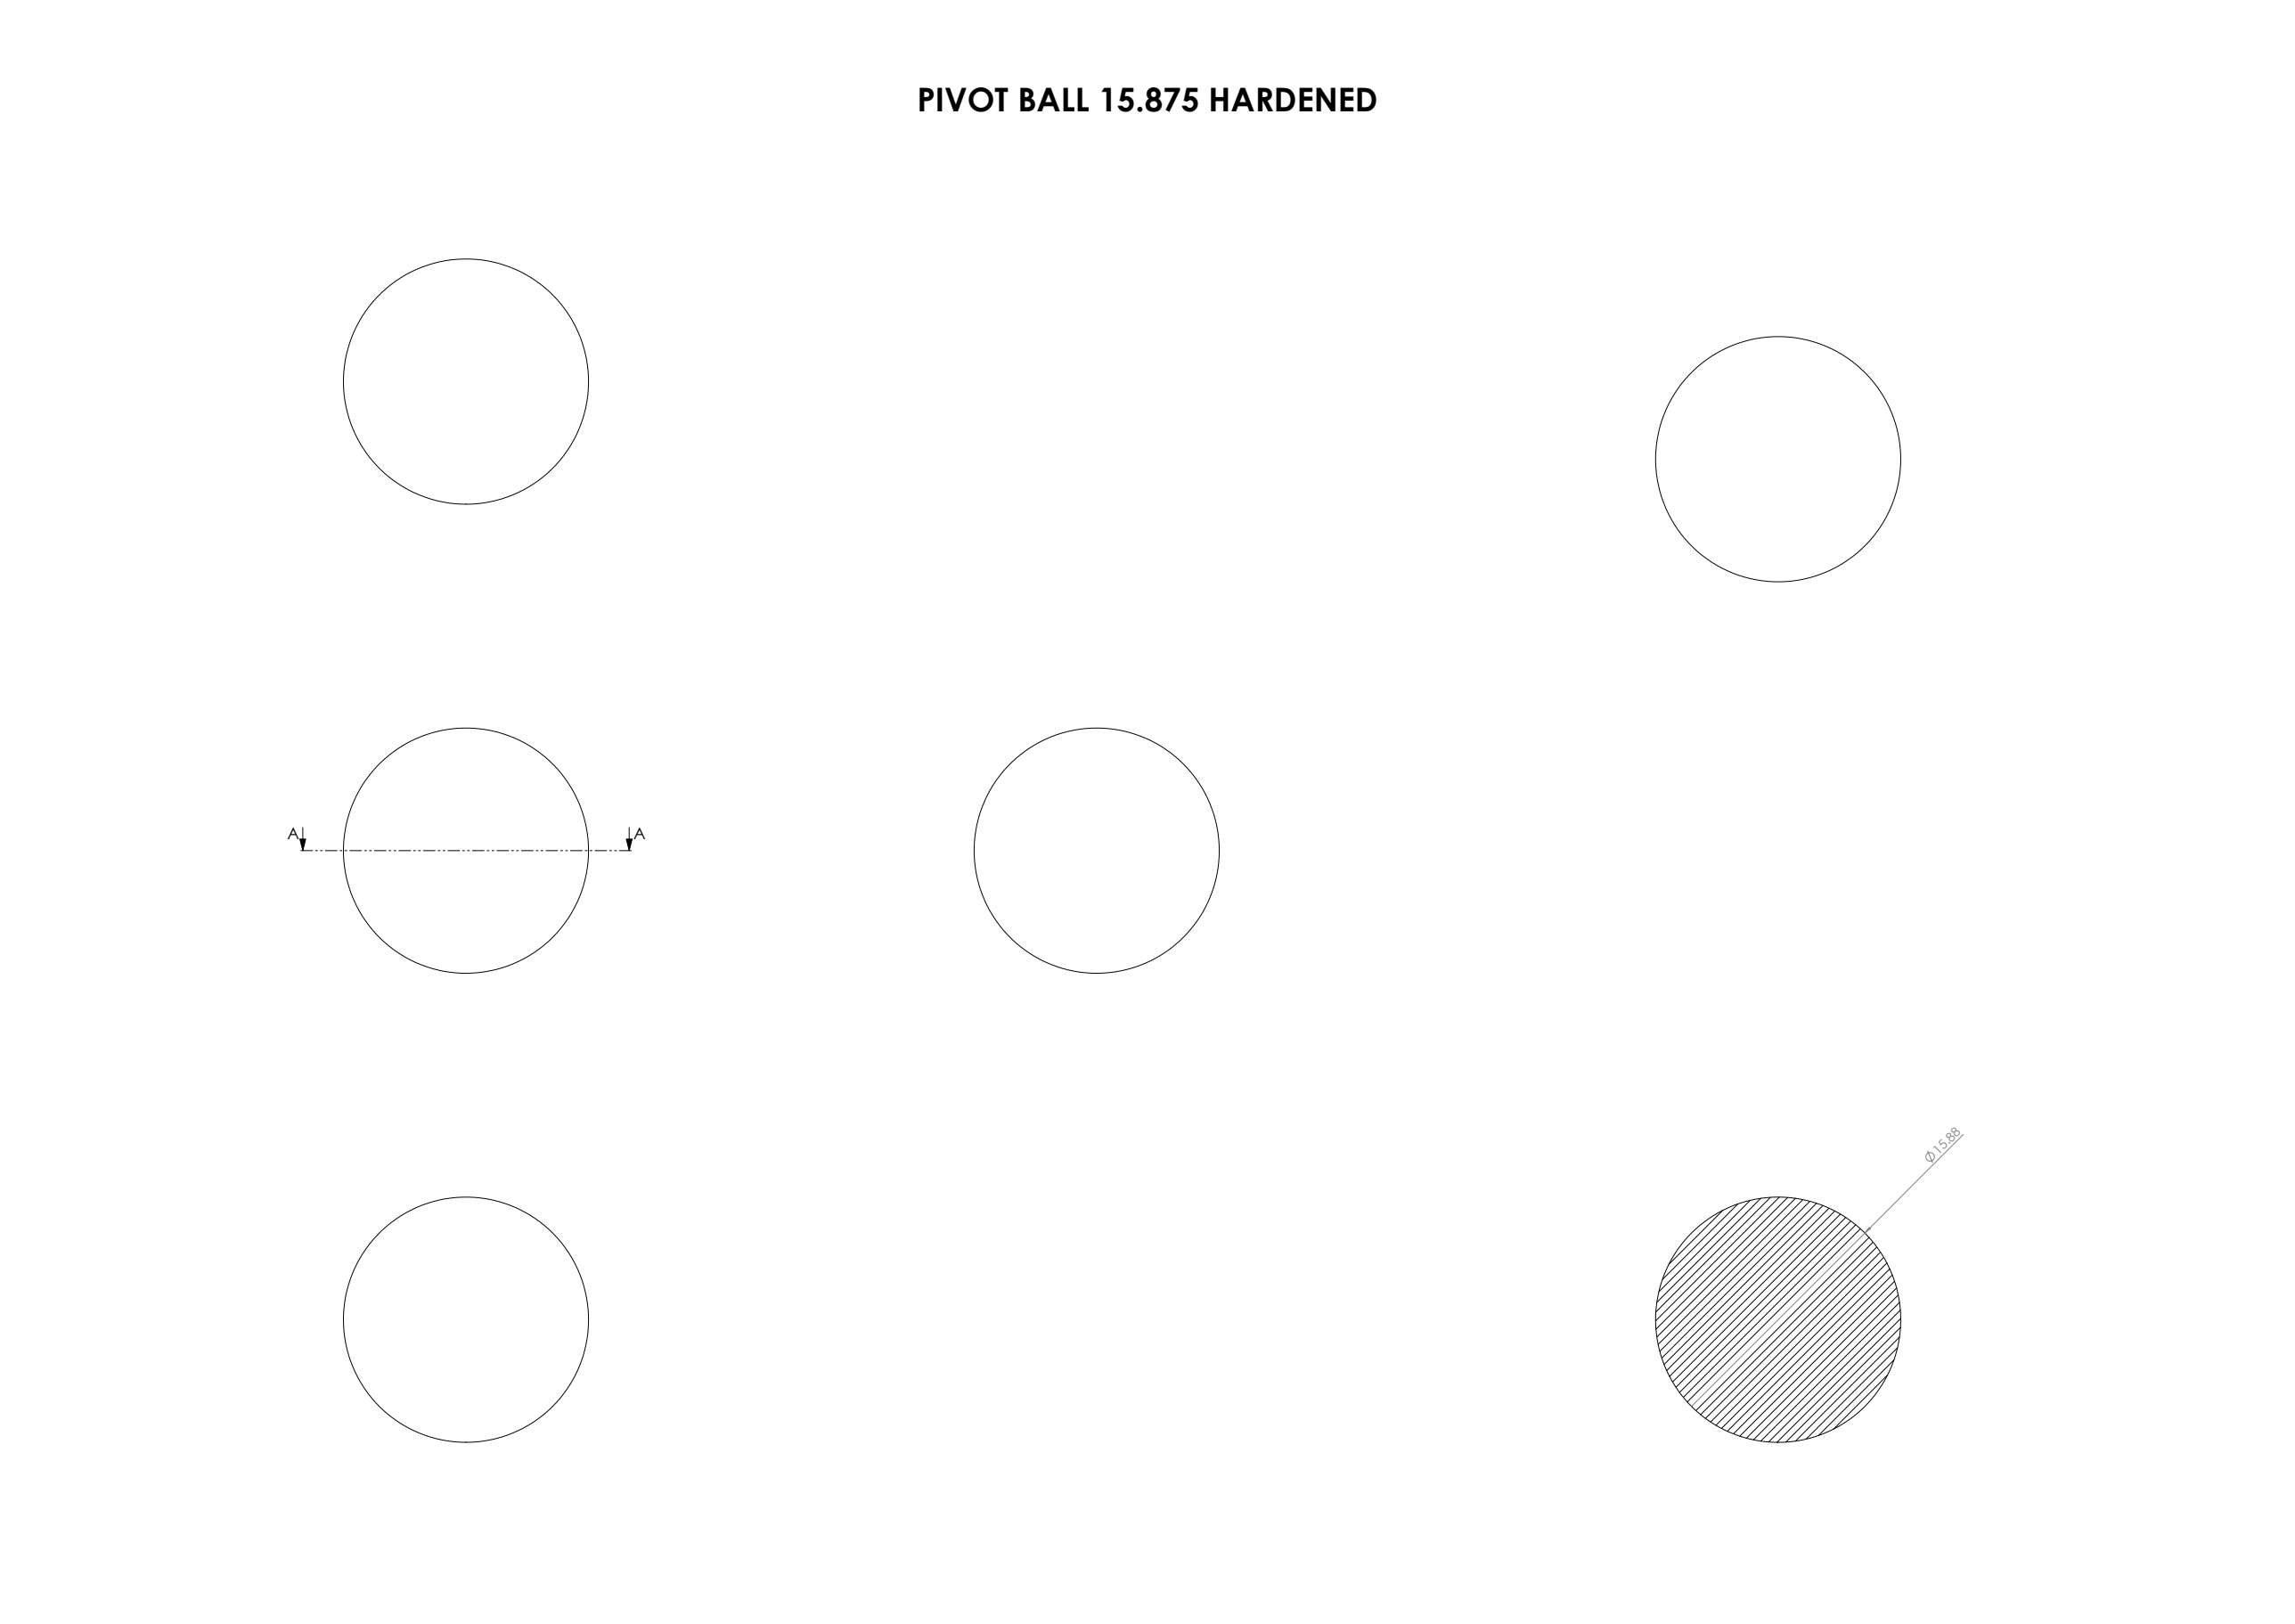
ISO-10303-21;
HEADER;
/* Generated by software containing ST-Developer
 * from STEP Tools, Inc. (www.steptools.com) 
 */

FILE_DESCRIPTION(
/* description */ (''),
/* implementation_level */ '2;1');

FILE_NAME(
/* name */ '09_Pivot_Ball_15.875_Hardened.step',
/* time_stamp */ '2026-10-21T01:56:51-07:00',
/* author */ (''),
/* organization */ (''),
/* preprocessor_version */ 'ST-DEVELOPER v20.2',
/* originating_system */ 'Autodesk Translation Framework v15.15.0.0',
/* authorisation */ '');

FILE_SCHEMA (('AUTOMOTIVE_DESIGN { 1 0 10303 214 3 1 1 }'));
ENDSEC;

DATA;
#10=MECHANICAL_DESIGN_GEOMETRIC_PRESENTATION_REPRESENTATION('',(#277),#82384);
#155=SPHERICAL_SURFACE('',#32076,7.9375);
#239=SHAPE_REPRESENTATION_RELATIONSHIP('SRR','None',#82473,#258);
#258=ADVANCED_BREP_SHAPE_REPRESENTATION('',(#296),#82372);
#277=STYLED_ITEM('',(#82624),#296);
#296=MANIFOLD_SOLID_BREP('Body1',#30668);
#1528=CIRCLE('',#32077,7.9375);
#4375=FACE_OUTER_BOUND('',#6333,.T.);
#6333=EDGE_LOOP('',(#23039,#23040));
#13179=VERTEX_POINT('',#48890);
#13180=VERTEX_POINT('',#48891);
#16741=EDGE_CURVE('',#13179,#13180,#1528,.T.);
#23039=ORIENTED_EDGE('',*,*,#16741,.T.);
#23040=ORIENTED_EDGE('',*,*,#16741,.F.);
#29703=ADVANCED_FACE('',(#4375),#155,.T.);
#30668=CLOSED_SHELL('',(#29703));
#32075=AXIS2_PLACEMENT_3D('',#48888,#36877,#36878);
#32076=AXIS2_PLACEMENT_3D('',#48889,#36879,#36880);
#32077=AXIS2_PLACEMENT_3D('',#48892,#36881,#36882);
#36877=DIRECTION('axis',(0.,0.,1.));
#36878=DIRECTION('refdir',(1.,0.,0.));
#36879=DIRECTION('center_axis',(6.12323399573677E-17,0.,1.));
#36880=DIRECTION('ref_axis',(1.,0.,0.));
#36881=DIRECTION('center_axis',(1.22464679914735E-16,-1.,0.));
#36882=DIRECTION('ref_axis',(-1.,-1.22464679914735E-16,0.));
#48888=CARTESIAN_POINT('',(0.,0.,0.));
#48889=CARTESIAN_POINT('Origin',(0.,0.,0.));
#48890=CARTESIAN_POINT('',(-4.86031698411606E-16,-5.95217163743925E-32,
7.9375));
#48891=CARTESIAN_POINT('',(-4.86031698411606E-16,-5.95217163743925E-32,
-7.9375));
#48892=CARTESIAN_POINT('Origin',(0.,0.,0.));
#82351=UNCERTAINTY_MEASURE_WITH_UNIT(LENGTH_MEASURE(0.01),#82385,
'DISTANCE_ACCURACY_VALUE',
'Maximum model space distance between geometric entities at asserted c
onnectivities');
#82363=UNCERTAINTY_MEASURE_WITH_UNIT(LENGTH_MEASURE(0.01),#82385,
'DISTANCE_ACCURACY_VALUE',
'Maximum model space distance between geometric entities at asserted c
onnectivities');
#82372=(
GEOMETRIC_REPRESENTATION_CONTEXT(3)
GLOBAL_UNCERTAINTY_ASSIGNED_CONTEXT((#82351))
GLOBAL_UNIT_ASSIGNED_CONTEXT((#82385,#82387,#82388))
REPRESENTATION_CONTEXT('','3D')
);
#82384=(
GEOMETRIC_REPRESENTATION_CONTEXT(3)
GLOBAL_UNCERTAINTY_ASSIGNED_CONTEXT((#82363))
GLOBAL_UNIT_ASSIGNED_CONTEXT((#82385,#82387,#82388))
REPRESENTATION_CONTEXT('','3D')
);
#82385=(
LENGTH_UNIT()
NAMED_UNIT(*)
SI_UNIT(.MILLI.,.METRE.)
);
#82387=(
NAMED_UNIT(*)
PLANE_ANGLE_UNIT()
SI_UNIT($,.RADIAN.)
);
#82388=(
NAMED_UNIT(*)
SI_UNIT($,.STERADIAN.)
SOLID_ANGLE_UNIT()
);
#82397=SHAPE_DEFINITION_REPRESENTATION(#82417,#82473);
#82417=PRODUCT_DEFINITION_SHAPE('',$,#82494);
#82473=SHAPE_REPRESENTATION('',(#32075),#82372);
#82485=PRODUCT_DEFINITION_CONTEXT('part definition',#82547,'design');
#82494=PRODUCT_DEFINITION('2026-10-20-12-38-19-717',
'09_Pivot_Ball_15.875_Hardened',#82514,#82485);
#82514=PRODUCT_DEFINITION_FORMATION('',$,#82557);
#82547=APPLICATION_CONTEXT(
'Core Data for Automotive Mechanical Design Process');
#82548=PRODUCT_CONTEXT('part definition',#82547,'mechanical');
#82557=PRODUCT('2026-10-20-12-38-19-717',
'09_Pivot_Ball_15.875_Hardened',$,(#82548));
#82618=COLOUR_RGB('Sky Blue',0.24,0.69,0.87);
#82619=FILL_AREA_STYLE_COLOUR('',#82618);
#82620=FILL_AREA_STYLE('',(#82619));
#82621=SURFACE_STYLE_FILL_AREA(#82620);
#82622=SURFACE_SIDE_STYLE('',(#82621));
#82623=SURFACE_STYLE_USAGE(.BOTH.,#82622);
#82624=PRESENTATION_STYLE_ASSIGNMENT((#82623));
ENDSEC;
END-ISO-10303-21;
